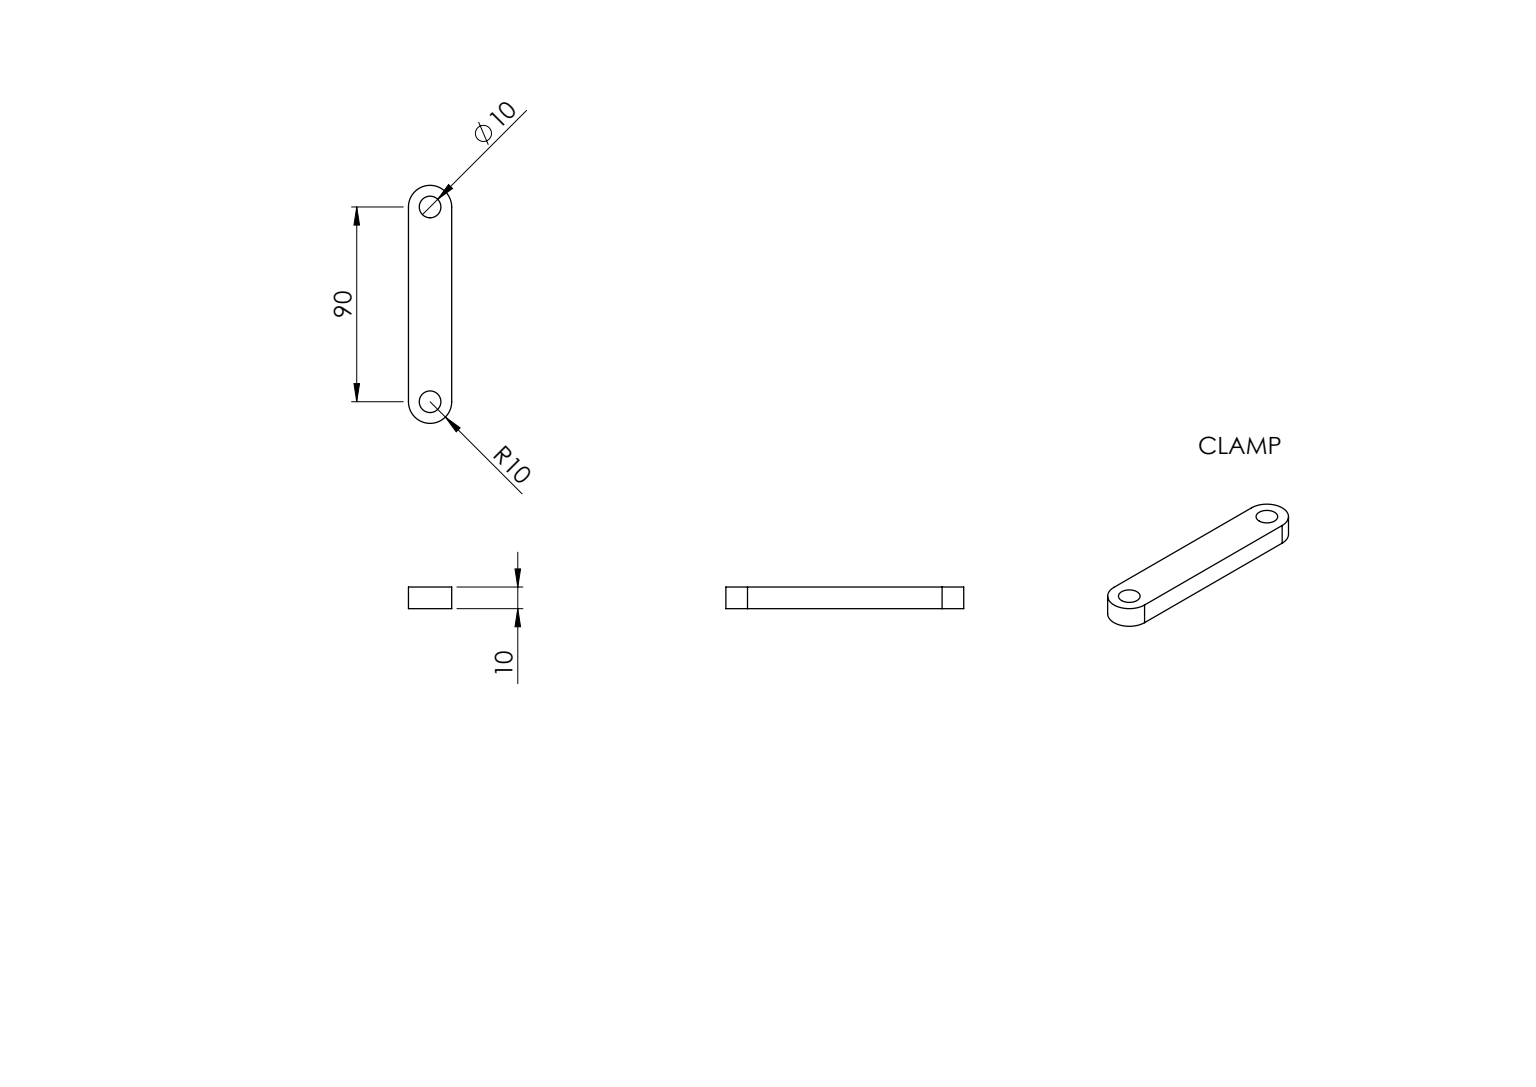
ISO-10303-21;
HEADER;
FILE_DESCRIPTION (('STEP AP214'),
    '1' );
FILE_NAME ('clamp.step',
    '2026-10-27T14:18:53',
    ( '' ),
    ( '' ),
    'SwSTEP 2.0',
    'SolidWorks 2026',
    '' );
FILE_SCHEMA (( 'AUTOMOTIVE_DESIGN' ));
ENDSEC;

DATA;
#13=EDGE_LOOP ( 'NONE', ( #5766, #2705, #5746, #232 ) ) ;
#85=ORIENTED_EDGE ( 'NONE', *, *, #3683, .T. ) ;
#87=DIRECTION ( 'NONE',  ( -0.000000000000000000, -1.000000000000000000, -0.000000000000000000 ) ) ;
#88=CIRCLE ( 'NONE', #5797, 5.000000000000004441 ) ;
#89=CARTESIAN_POINT ( 'NONE',  ( -55.00000000000001421, 40.00000000000000000, -45.00000000000000000 ) ) ;
#105=VERTEX_POINT ( 'NONE', #4634 ) ;
#111=VERTEX_POINT ( 'NONE', #3686 ) ;
#120=FACE_BOUND ( 'NONE', #3180, .T. ) ;
#147=CLOSED_SHELL ( 'NONE', ( #248, #2661, #5068, #1341, #3720, #5571, #3327, #1429, #4479, #1422, #4024 ) ) ;
#150=DIRECTION ( 'NONE',  ( 0.000000000000000000, 1.000000000000000000, 0.000000000000000000 ) ) ;
#188=STYLED_ITEM('',(#6006),#2182);
#203=EDGE_CURVE ( 'NONE', #1147, #2495, #5910, .T. ) ;
#217=ORIENTED_EDGE ( 'NONE', *, *, #5542, .F. ) ;
#232=ORIENTED_EDGE ( 'NONE', *, *, #1791, .F. ) ;
#234=DIRECTION ( 'NONE',  ( 0.000000000000000000, 1.000000000000000000, 0.000000000000000000 ) ) ;
#248=ADVANCED_FACE ( 'NONE', ( #4015 ), #1620, .F. ) ;
#256=APPLICATION_CONTEXT ( 'automotive_design' ) ;
#258=ORIENTED_EDGE ( 'NONE', *, *, #3702, .T. ) ;
#270=DIRECTION ( 'NONE',  ( -0.000000000000000000, -1.000000000000000000, -0.000000000000000000 ) ) ;
#325=CARTESIAN_POINT ( 'NONE',  ( -45.00000000000001421, 30.00000000000000355, -50.00000000000000000 ) ) ;
#340=LINE ( 'NONE', #5874, #5255 ) ;
#355=CARTESIAN_POINT ( 'NONE',  ( -45.00000000000001421, 40.00000000000000000, 50.00000000000000000 ) ) ;
#361=AXIS2_PLACEMENT_3D ( 'NONE', #2845, #4273, #538 ) ;
#367=EDGE_CURVE ( 'NONE', #1773, #5556, #4512, .T. ) ;
#377=VERTEX_POINT ( 'NONE', #441 ) ;
#417=VECTOR ( 'NONE', #1999, 1000.000000000000000 ) ;
#441=CARTESIAN_POINT ( 'NONE',  ( -45.00000000000001421, 40.00000000000000000, 50.00000000000000000 ) ) ;
#531=EDGE_CURVE ( 'NONE', #1773, #105, #641, .T. ) ;
#538=DIRECTION ( 'NONE',  ( 0.000000000000000000, 0.000000000000000000, -1.000000000000000000 ) ) ;
#569=ORIENTED_EDGE ( 'NONE', *, *, #1573, .F. ) ;
#596=PRODUCT_CONTEXT ( 'NONE', #256, 'mechanical' ) ;
#608=( NAMED_UNIT ( * ) PLANE_ANGLE_UNIT ( ) SI_UNIT ( $, .RADIAN. ) );
#625=DIRECTION ( 'NONE',  ( -0.000000000000000000, -1.000000000000000000, -0.000000000000000000 ) ) ;
#641=LINE ( 'NONE', #2484, #4530 ) ;
#649=DIRECTION ( 'NONE',  ( 0.000000000000000000, 0.000000000000000000, 1.000000000000000000 ) ) ;
#657=DIRECTION ( 'NONE',  ( 0.000000000000000000, 0.000000000000000000, 1.000000000000000000 ) ) ;
#667=DIRECTION ( 'NONE',  ( 1.000000000000000000, 0.000000000000000000, 0.000000000000000000 ) ) ;
#716=CARTESIAN_POINT ( 'NONE',  ( -45.00000000000001421, 40.00000000000000000, -55.00000000000000000 ) ) ;
#719=EDGE_CURVE ( 'NONE', #4755, #3109, #5913, .T. ) ;
#720=CARTESIAN_POINT ( 'NONE',  ( -45.00000000000001421, 40.00000000000000000, -45.00000000000000000 ) ) ;
#739=ORIENTED_EDGE ( 'NONE', *, *, #1238, .F. ) ;
#747=PLANE ( 'NONE',  #3499 ) ;
#791=PRODUCT_DEFINITION ( 'UNKNOWN', '', #4303, #1117 ) ;
#796=EDGE_LOOP ( 'NONE', ( #4911, #5822 ) ) ;
#813=CARTESIAN_POINT ( 'NONE',  ( -35.00000000000000711, 30.00000000000000355, 45.00000000000000000 ) ) ;
#840=DIRECTION ( 'NONE',  ( 0.000000000000000000, 1.000000000000000000, 0.000000000000000000 ) ) ;
#842=DIRECTION ( 'NONE',  ( 0.000000000000000000, 0.000000000000000000, -1.000000000000000000 ) ) ;
#858=CARTESIAN_POINT ( 'NONE',  ( -45.00000000000001421, 40.00000000000000000, 45.00000000000000000 ) ) ;
#869=FACE_OUTER_BOUND ( 'NONE', #5036, .T. ) ;
#908=DIRECTION ( 'NONE',  ( 0.000000000000000000, 0.000000000000000000, 1.000000000000000000 ) ) ;
#939=VERTEX_POINT ( 'NONE', #5636 ) ;
#955=ORIENTED_EDGE ( 'NONE', *, *, #1985, .T. ) ;
#956=MECHANICAL_DESIGN_GEOMETRIC_PRESENTATION_REPRESENTATION('',(#188),#1645);
#995=FACE_OUTER_BOUND ( 'NONE', #13, .T. ) ;
#996=DIRECTION ( 'NONE',  ( 0.000000000000000000, 0.000000000000000000, 1.000000000000000000 ) ) ;
#1011=ORIENTED_EDGE ( 'NONE', *, *, #1756, .T. ) ;
#1018=EDGE_LOOP ( 'NONE', ( #5388, #1028, #3124, #4232 ) ) ;
#1028=ORIENTED_EDGE ( 'NONE', *, *, #5949, .F. ) ;
#1048=ORIENTED_EDGE ( 'NONE', *, *, #3427, .F. ) ;
#1057=AXIS2_PLACEMENT_3D ( 'NONE', #1923, #4598, #1476 ) ;
#1101=FACE_OUTER_BOUND ( 'NONE', #4420, .T. ) ;
#1113=SHAPE_REPRESENTATION ( 'clamp', ( #5080 ), #4776 ) ;
#1116=UNCERTAINTY_MEASURE_WITH_UNIT (LENGTH_MEASURE( 1.000000000000000082E-05 ), #1219, 'distance_accuracy_value', 'NONE');
#1117=PRODUCT_DEFINITION_CONTEXT ( 'detailed design', #5329, 'design' ) ;
#1120=EDGE_CURVE ( 'NONE', #3568, #3307, #2068, .T. ) ;
#1134=LINE ( 'NONE', #2938, #3781 ) ;
#1147=VERTEX_POINT ( 'NONE', #4828 ) ;
#1159=AXIS2_PLACEMENT_3D ( 'NONE', #3827, #1520, #5224 ) ;
#1190=( NAMED_UNIT ( * ) SI_UNIT ( $, .STERADIAN. ) SOLID_ANGLE_UNIT ( ) );
#1193=DIRECTION ( 'NONE',  ( -1.000000000000000000, 0.000000000000000000, 0.000000000000000000 ) ) ;
#1215=CARTESIAN_POINT ( 'NONE',  ( -55.00000000000001421, 30.00000000000000355, -45.00000000000000000 ) ) ;
#1219=( LENGTH_UNIT ( ) NAMED_UNIT ( * ) SI_UNIT ( .MILLI., .METRE. ) );
#1222=CARTESIAN_POINT ( 'NONE',  ( -35.00000000000000711, 40.00000000000000000, 45.00000000000000000 ) ) ;
#1230=CARTESIAN_POINT ( 'NONE',  ( -45.00000000000001421, 30.00000000000000355, -45.00000000000000000 ) ) ;
#1238=EDGE_CURVE ( 'NONE', #3109, #3549, #5477, .T. ) ;
#1257=ORIENTED_EDGE ( 'NONE', *, *, #1573, .T. ) ;
#1273=VECTOR ( 'NONE', #2528, 1000.000000000000000 ) ;
#1276=FILL_AREA_STYLE ('',( #3580 ) ) ;
#1287=EDGE_CURVE ( 'NONE', #2495, #4600, #3639, .T. ) ;
#1298=DIRECTION ( 'NONE',  ( -0.000000000000000000, -1.000000000000000000, -0.000000000000000000 ) ) ;
#1301=CARTESIAN_POINT ( 'NONE',  ( -45.00000000000001421, 40.00000000000000000, 45.00000000000000000 ) ) ;
#1341=ADVANCED_FACE ( 'NONE', ( #2873, #5209, #120 ), #1898, .T. ) ;
#1349=DIRECTION ( 'NONE',  ( 0.000000000000000000, 1.000000000000000000, 0.000000000000000000 ) ) ;
#1358=ORIENTED_EDGE ( 'NONE', *, *, #203, .T. ) ;
#1362=DIRECTION ( 'NONE',  ( -0.000000000000000000, -0.000000000000000000, 1.000000000000000000 ) ) ;
#1368=AXIS2_PLACEMENT_3D ( 'NONE', #858, #3655, #4231 ) ;
#1380=VECTOR ( 'NONE', #2853, 1000.000000000000000 ) ;
#1418=CIRCLE ( 'NONE', #2117, 10.00000000000000178 ) ;
#1422=ADVANCED_FACE ( 'NONE', ( #995 ), #3810, .F. ) ;
#1425=CARTESIAN_POINT ( 'NONE',  ( -45.00000000000001421, 40.00000000000000000, -45.00000000000000000 ) ) ;
#1429=ADVANCED_FACE ( 'NONE', ( #2386 ), #1532, .T. ) ;
#1476=DIRECTION ( 'NONE',  ( 0.000000000000000000, 0.000000000000000000, -1.000000000000000000 ) ) ;
#1493=ORIENTED_EDGE ( 'NONE', *, *, #1238, .T. ) ;
#1495=AXIS2_PLACEMENT_3D ( 'NONE', #1301, #2761, #908 ) ;
#1520=DIRECTION ( 'NONE',  ( 0.000000000000000000, 1.000000000000000000, 0.000000000000000000 ) ) ;
#1532=CYLINDRICAL_SURFACE ( 'NONE', #5018, 10.00000000000000178 ) ;
#1559=CIRCLE ( 'NONE', #5347, 10.00000000000000178 ) ;
#1573=EDGE_CURVE ( 'NONE', #939, #3970, #2780, .T. ) ;
#1607=UNCERTAINTY_MEASURE_WITH_UNIT (LENGTH_MEASURE( 1.000000000000000082E-05 ), #5602, 'distance_accuracy_value', 'NONE');
#1609=ORIENTED_EDGE ( 'NONE', *, *, #4675, .T. ) ;
#1620=CYLINDRICAL_SURFACE ( 'NONE', #5826, 5.000000000000004441 ) ;
#1633=DIRECTION ( 'NONE',  ( 0.000000000000000000, 0.000000000000000000, 1.000000000000000000 ) ) ;
#1638=DIRECTION ( 'NONE',  ( 0.000000000000000000, 0.000000000000000000, 1.000000000000000000 ) ) ;
#1640=AXIS2_PLACEMENT_3D ( 'NONE', #1230, #1744, #3085 ) ;
#1645=( GEOMETRIC_REPRESENTATION_CONTEXT ( 3 ) GLOBAL_UNCERTAINTY_ASSIGNED_CONTEXT ( ( #1116 ) ) GLOBAL_UNIT_ASSIGNED_CONTEXT ( ( #1219, #1735, #1190 ) ) REPRESENTATION_CONTEXT ( 'NONE', 'WORKASPACE' ) );
#1657=AXIS2_PLACEMENT_3D ( 'NONE', #3859, #1193, #2931 ) ;
#1658=EDGE_LOOP ( 'NONE', ( #1048, #3597, #2673, #5918 ) ) ;
#1659=EDGE_CURVE ( 'NONE', #111, #377, #88, .T. ) ;
#1663=DIRECTION ( 'NONE',  ( 0.000000000000000000, 0.000000000000000000, 1.000000000000000000 ) ) ;
#1683=ORIENTED_EDGE ( 'NONE', *, *, #3427, .T. ) ;
#1691=CARTESIAN_POINT ( 'NONE',  ( -35.00000000000000711, 40.00000000000000000, -45.00000000000000000 ) ) ;
#1694=DIRECTION ( 'NONE',  ( -0.000000000000000000, -1.000000000000000000, -0.000000000000000000 ) ) ;
#1723=EDGE_CURVE ( 'NONE', #3307, #3568, #2735, .T. ) ;
#1735=( NAMED_UNIT ( * ) PLANE_ANGLE_UNIT ( ) SI_UNIT ( $, .RADIAN. ) );
#1744=DIRECTION ( 'NONE',  ( 0.000000000000000000, 1.000000000000000000, 0.000000000000000000 ) ) ;
#1748=CYLINDRICAL_SURFACE ( 'NONE', #3511, 10.00000000000000178 ) ;
#1756=EDGE_CURVE ( 'NONE', #5556, #4755, #1418, .T. ) ;
#1773=VERTEX_POINT ( 'NONE', #1691 ) ;
#1786=ORIENTED_EDGE ( 'NONE', *, *, #203, .F. ) ;
#1791=EDGE_CURVE ( 'NONE', #3262, #2126, #4120, .T. ) ;
#1811=EDGE_LOOP ( 'NONE', ( #569, #4895 ) ) ;
#1853=DIRECTION ( 'NONE',  ( 0.000000000000000000, 0.000000000000000000, 1.000000000000000000 ) ) ;
#1898=PLANE ( 'NONE',  #5578 ) ;
#1915=CARTESIAN_POINT ( 'NONE',  ( -55.00000000000001421, 40.00000000000000000, 45.00000000000000000 ) ) ;
#1921=DIRECTION ( 'NONE',  ( 0.000000000000000000, 0.000000000000000000, -1.000000000000000000 ) ) ;
#1923=CARTESIAN_POINT ( 'NONE',  ( -45.00000000000001421, 40.00000000000000000, -45.00000000000000000 ) ) ;
#1927=PRODUCT ( 'clamp', 'clamp', '', ( #596 ) ) ;
#1929=( NAMED_UNIT ( * ) SI_UNIT ( $, .STERADIAN. ) SOLID_ANGLE_UNIT ( ) );
#1985=EDGE_CURVE ( 'NONE', #4600, #2954, #2800, .T. ) ;
#1999=DIRECTION ( 'NONE',  ( -0.000000000000000000, -1.000000000000000000, -0.000000000000000000 ) ) ;
#2008=PLANE ( 'NONE',  #1657 ) ;
#2011=EDGE_LOOP ( 'NONE', ( #5869, #5688, #1358, #5895 ) ) ;
#2014=FACE_BOUND ( 'NONE', #796, .T. ) ;
#2033=ORIENTED_EDGE ( 'NONE', *, *, #4675, .F. ) ;
#2054=( GEOMETRIC_REPRESENTATION_CONTEXT ( 3 ) GLOBAL_UNCERTAINTY_ASSIGNED_CONTEXT ( ( #1607 ) ) GLOBAL_UNIT_ASSIGNED_CONTEXT ( ( #5602, #608, #1929 ) ) REPRESENTATION_CONTEXT ( 'NONE', 'WORKASPACE' ) );
#2055=CARTESIAN_POINT ( 'NONE',  ( -55.00000000000001421, 30.00000000000000355, 45.00000000000000000 ) ) ;
#2068=CIRCLE ( 'NONE', #2945, 5.000000000000004441 ) ;
#2082=FACE_BOUND ( 'NONE', #2783, .T. ) ;
#2085=DIRECTION ( 'NONE',  ( 0.000000000000000000, 1.000000000000000000, 0.000000000000000000 ) ) ;
#2117=AXIS2_PLACEMENT_3D ( 'NONE', #3634, #840, #2175 ) ;
#2126=VERTEX_POINT ( 'NONE', #325 ) ;
#2139=VECTOR ( 'NONE', #3110, 1000.000000000000000 ) ;
#2143=CARTESIAN_POINT ( 'NONE',  ( -55.00000000000001421, 40.00000000000000000, -45.00000000000000000 ) ) ;
#2154=COLOUR_RGB ( '',0.8941176470588234615, 0.8941176470588234615, 0.8941176470588234615 ) ;
#2175=DIRECTION ( 'NONE',  ( 0.000000000000000000, 0.000000000000000000, 1.000000000000000000 ) ) ;
#2182=MANIFOLD_SOLID_BREP ( 'Boss-Extrude1', #147 ) ;
#2185=( NAMED_UNIT ( * ) PLANE_ANGLE_UNIT ( ) SI_UNIT ( $, .RADIAN. ) );
#2221=LINE ( 'NONE', #355, #2139 ) ;
#2229=DIRECTION ( 'NONE',  ( 0.000000000000000000, 0.000000000000000000, 1.000000000000000000 ) ) ;
#2342=MECHANICAL_DESIGN_GEOMETRIC_PRESENTATION_REPRESENTATION('',(#5551),#2054);
#2386=FACE_OUTER_BOUND ( 'NONE', #5197, .T. ) ;
#2437=AXIS2_PLACEMENT_3D ( 'NONE', #5011, #5511, #2718 ) ;
#2452=EDGE_LOOP ( 'NONE', ( #5202, #4313, #1786, #5741, #3673 ) ) ;
#2468=LINE ( 'NONE', #3416, #4285 ) ;
#2484=CARTESIAN_POINT ( 'NONE',  ( -35.00000000000000711, 40.00000000000000000, -45.00000000000000000 ) ) ;
#2494=FACE_OUTER_BOUND ( 'NONE', #2011, .T. ) ;
#2495=VERTEX_POINT ( 'NONE', #1215 ) ;
#2528=DIRECTION ( 'NONE',  ( 0.000000000000000000, 0.000000000000000000, -1.000000000000000000 ) ) ;
#2538=DIRECTION ( 'NONE',  ( 0.000000000000000000, 0.000000000000000000, -1.000000000000000000 ) ) ;
#2613=CARTESIAN_POINT ( 'NONE',  ( -45.00000000000001421, 40.00000000000000000, 45.00000000000000000 ) ) ;
#2641=AXIS2_PLACEMENT_3D ( 'NONE', #4733, #5664, #5632 ) ;
#2661=ADVANCED_FACE ( 'NONE', ( #5210 ), #2904, .F. ) ;
#2673=ORIENTED_EDGE ( 'NONE', *, *, #5542, .T. ) ;
#2696=DIRECTION ( 'NONE',  ( -0.000000000000000000, -0.000000000000000000, 1.000000000000000000 ) ) ;
#2705=ORIENTED_EDGE ( 'NONE', *, *, #2725, .T. ) ;
#2718=DIRECTION ( 'NONE',  ( 0.000000000000000000, 0.000000000000000000, 1.000000000000000000 ) ) ;
#2725=EDGE_CURVE ( 'NONE', #3970, #939, #4851, .T. ) ;
#2735=CIRCLE ( 'NONE', #2437, 5.000000000000004441 ) ;
#2761=DIRECTION ( 'NONE',  ( 0.000000000000000000, 1.000000000000000000, 0.000000000000000000 ) ) ;
#2780=CIRCLE ( 'NONE', #3556, 5.000000000000004441 ) ;
#2783=EDGE_LOOP ( 'NONE', ( #1609, #3056 ) ) ;
#2791=EDGE_CURVE ( 'NONE', #4755, #2495, #4562, .T. ) ;
#2800=CIRCLE ( 'NONE', #5416, 10.00000000000000178 ) ;
#2845=CARTESIAN_POINT ( 'NONE',  ( -45.00000000000001421, 40.00000000000000000, -45.00000000000000000 ) ) ;
#2853=DIRECTION ( 'NONE',  ( -0.000000000000000000, -1.000000000000000000, -0.000000000000000000 ) ) ;
#2873=FACE_BOUND ( 'NONE', #1811, .T. ) ;
#2896=CARTESIAN_POINT ( 'NONE',  ( -45.00000000000001421, 40.00000000000000000, -45.00000000000000000 ) ) ;
#2904=CYLINDRICAL_SURFACE ( 'NONE', #1057, 5.000000000000004441 ) ;
#2910=PRESENTATION_STYLE_ASSIGNMENT (( #4767 ) ) ;
#2931=DIRECTION ( 'NONE',  ( 0.000000000000000000, 0.000000000000000000, 1.000000000000000000 ) ) ;
#2938=CARTESIAN_POINT ( 'NONE',  ( -35.00000000000000711, 40.00000000000000000, 45.00000000000000000 ) ) ;
#2945=AXIS2_PLACEMENT_3D ( 'NONE', #4949, #3938, #1638 ) ;
#2954=VERTEX_POINT ( 'NONE', #813 ) ;
#2955=ORIENTED_EDGE ( 'NONE', *, *, #531, .F. ) ;
#2994=VECTOR ( 'NONE', #1362, 1000.000000000000000 ) ;
#2995=CARTESIAN_POINT ( 'NONE',  ( -45.00000000000001421, 30.00000000000000355, -45.00000000000000000 ) ) ;
#3006=VECTOR ( 'NONE', #3197, 1000.000000000000000 ) ;
#3021=CARTESIAN_POINT ( 'NONE',  ( -45.00000000000001421, 30.00000000000000355, -39.99999999999999289 ) ) ;
#3022=CARTESIAN_POINT ( 'NONE',  ( -45.00000000000001421, 40.00000000000000000, 45.00000000000000000 ) ) ;
#3056=ORIENTED_EDGE ( 'NONE', *, *, #1791, .T. ) ;
#3068=CARTESIAN_POINT ( 'NONE',  ( -45.00000000000001421, 40.00000000000000000, -39.99999999999999289 ) ) ;
#3075=ORIENTED_EDGE ( 'NONE', *, *, #1659, .T. ) ;
#3085=DIRECTION ( 'NONE',  ( 0.000000000000000000, 0.000000000000000000, 1.000000000000000000 ) ) ;
#3109=VERTEX_POINT ( 'NONE', #1915 ) ;
#3110=DIRECTION ( 'NONE',  ( -0.000000000000000000, -1.000000000000000000, -0.000000000000000000 ) ) ;
#3124=ORIENTED_EDGE ( 'NONE', *, *, #719, .F. ) ;
#3126=AXIS2_PLACEMENT_3D ( 'NONE', #3022, #4880, #3508 ) ;
#3135=SURFACE_STYLE_FILL_AREA ( #1276 ) ;
#3180=EDGE_LOOP ( 'NONE', ( #4513, #3847 ) ) ;
#3195=( NAMED_UNIT ( * ) SI_UNIT ( $, .STERADIAN. ) SOLID_ANGLE_UNIT ( ) );
#3197=DIRECTION ( 'NONE',  ( -0.000000000000000000, -1.000000000000000000, -0.000000000000000000 ) ) ;
#3215=CARTESIAN_POINT ( 'NONE',  ( -45.00000000000001421, 40.00000000000000000, 45.00000000000000000 ) ) ;
#3257=CARTESIAN_POINT ( 'NONE',  ( -55.00000000000001421, 40.00000000000000000, 45.00000000000000000 ) ) ;
#3262=VERTEX_POINT ( 'NONE', #3021 ) ;
#3303=DIRECTION ( 'NONE',  ( 0.000000000000000000, 1.000000000000000000, 0.000000000000000000 ) ) ;
#3307=VERTEX_POINT ( 'NONE', #5361 ) ;
#3327=ADVANCED_FACE ( 'NONE', ( #1101 ), #2008, .F. ) ;
#3362=CARTESIAN_POINT ( 'NONE',  ( -45.00000000000001421, 40.00000000000000000, -45.00000000000000000 ) ) ;
#3416=CARTESIAN_POINT ( 'NONE',  ( -45.00000000000001421, 40.00000000000000000, -50.00000000000000000 ) ) ;
#3427=EDGE_CURVE ( 'NONE', #377, #3307, #2221, .T. ) ;
#3499=AXIS2_PLACEMENT_3D ( 'NONE', #4308, #150, #3838 ) ;
#3504=AXIS2_PLACEMENT_3D ( 'NONE', #2896, #4786, #4816 ) ;
#3508=DIRECTION ( 'NONE',  ( 0.000000000000000000, 0.000000000000000000, -1.000000000000000000 ) ) ;
#3511=AXIS2_PLACEMENT_3D ( 'NONE', #4430, #270, #842 ) ;
#3516=CARTESIAN_POINT ( 'NONE',  ( -35.00000000000000711, 40.00000000000000000, 45.00000000000000000 ) ) ;
#3527=CARTESIAN_POINT ( 'NONE',  ( 0.000000000000000000, 0.000000000000000000, 0.000000000000000000 ) ) ;
#3549=VERTEX_POINT ( 'NONE', #1222 ) ;
#3556=AXIS2_PLACEMENT_3D ( 'NONE', #720, #5811, #657 ) ;
#3565=CARTESIAN_POINT ( 'NONE',  ( -45.00000000000001421, 40.00000000000000000, -39.99999999999999289 ) ) ;
#3568=VERTEX_POINT ( 'NONE', #4608 ) ;
#3580=FILL_AREA_STYLE_COLOUR ( '', #2154 ) ;
#3597=ORIENTED_EDGE ( 'NONE', *, *, #4048, .T. ) ;
#3599=VECTOR ( 'NONE', #625, 1000.000000000000000 ) ;
#3634=CARTESIAN_POINT ( 'NONE',  ( -45.00000000000001421, 40.00000000000000000, -45.00000000000000000 ) ) ;
#3639=LINE ( 'NONE', #4057, #5461 ) ;
#3655=DIRECTION ( 'NONE',  ( 0.000000000000000000, 1.000000000000000000, 0.000000000000000000 ) ) ;
#3673=ORIENTED_EDGE ( 'NONE', *, *, #3755, .F. ) ;
#3683=EDGE_CURVE ( 'NONE', #3549, #1773, #1134, .T. ) ;
#3686=CARTESIAN_POINT ( 'NONE',  ( -45.00000000000001421, 40.00000000000000000, 39.99999999999999289 ) ) ;
#3702=EDGE_CURVE ( 'NONE', #105, #1147, #1559, .T. ) ;
#3720=ADVANCED_FACE ( 'NONE', ( #4917, #2082, #2014 ), #747, .F. ) ;
#3755=EDGE_CURVE ( 'NONE', #2954, #105, #5711, .T. ) ;
#3778=PLANE ( 'NONE',  #2641 ) ;
#3781=VECTOR ( 'NONE', #2538, 1000.000000000000000 ) ;
#3789=ORIENTED_EDGE ( 'NONE', *, *, #3683, .F. ) ;
#3803=ORIENTED_EDGE ( 'NONE', *, *, #4249, .T. ) ;
#3807=LINE ( 'NONE', #716, #3599 ) ;
#3810=CYLINDRICAL_SURFACE ( 'NONE', #361, 5.000000000000004441 ) ;
#3814=ORIENTED_EDGE ( 'NONE', *, *, #5105, .F. ) ;
#3826=EDGE_CURVE ( 'NONE', #939, #2126, #2468, .T. ) ;
#3827=CARTESIAN_POINT ( 'NONE',  ( -45.00000000000001421, 30.00000000000000355, -45.00000000000000000 ) ) ;
#3838=DIRECTION ( 'NONE',  ( 0.000000000000000000, -0.000000000000000000, 1.000000000000000000 ) ) ;
#3847=ORIENTED_EDGE ( 'NONE', *, *, #4048, .F. ) ;
#3859=CARTESIAN_POINT ( 'NONE',  ( -35.00000000000000711, 40.00000000000000000, 45.00000000000000000 ) ) ;
#3938=DIRECTION ( 'NONE',  ( 0.000000000000000000, 1.000000000000000000, 0.000000000000000000 ) ) ;
#3954=FACE_OUTER_BOUND ( 'NONE', #1658, .T. ) ;
#3970=VERTEX_POINT ( 'NONE', #3565 ) ;
#4015=FACE_OUTER_BOUND ( 'NONE', #4948, .T. ) ;
#4024=ADVANCED_FACE ( 'NONE', ( #3954 ), #5807, .F. ) ;
#4028=CARTESIAN_POINT ( 'NONE',  ( -45.00000000000001421, 40.00000000000000000, -55.00000000000000000 ) ) ;
#4048=EDGE_CURVE ( 'NONE', #377, #111, #5733, .T. ) ;
#4057=CARTESIAN_POINT ( 'NONE',  ( -55.00000000000001421, 30.00000000000000355, 45.00000000000000000 ) ) ;
#4120=CIRCLE ( 'NONE', #1640, 5.000000000000004441 ) ;
#4219=DIRECTION ( 'NONE',  ( 0.000000000000000000, 1.000000000000000000, 0.000000000000000000 ) ) ;
#4222=PRODUCT_DEFINITION_SHAPE ( 'NONE', 'NONE',  #791 ) ;
#4223=ORIENTED_EDGE ( 'NONE', *, *, #367, .F. ) ;
#4231=DIRECTION ( 'NONE',  ( 0.000000000000000000, 0.000000000000000000, 1.000000000000000000 ) ) ;
#4232=ORIENTED_EDGE ( 'NONE', *, *, #2791, .T. ) ;
#4249=EDGE_CURVE ( 'NONE', #3970, #3262, #4900, .T. ) ;
#4263=ORIENTED_EDGE ( 'NONE', *, *, #5574, .T. ) ;
#4273=DIRECTION ( 'NONE',  ( -0.000000000000000000, -1.000000000000000000, -0.000000000000000000 ) ) ;
#4285=VECTOR ( 'NONE', #4332, 1000.000000000000000 ) ;
#4288=LINE ( 'NONE', #4739, #1380 ) ;
#4302=CARTESIAN_POINT ( 'NONE',  ( -35.00000000000000711, 30.00000000000000355, 45.00000000000000000 ) ) ;
#4303=PRODUCT_DEFINITION_FORMATION_WITH_SPECIFIED_SOURCE ( 'ANY', '', #1927, .NOT_KNOWN. ) ;
#4306=SHAPE_DEFINITION_REPRESENTATION ( #4222, #1113 ) ;
#4308=CARTESIAN_POINT ( 'NONE',  ( -45.00000000000001421, 30.00000000000000355, 45.00000000000000000 ) ) ;
#4313=ORIENTED_EDGE ( 'NONE', *, *, #1287, .F. ) ;
#4330=ORIENTED_EDGE ( 'NONE', *, *, #5574, .F. ) ;
#4332=DIRECTION ( 'NONE',  ( -0.000000000000000000, -1.000000000000000000, -0.000000000000000000 ) ) ;
#4376=CIRCLE ( 'NONE', #4875, 5.000000000000004441 ) ;
#4420=EDGE_LOOP ( 'NONE', ( #5901, #2955, #3789, #4263 ) ) ;
#4430=CARTESIAN_POINT ( 'NONE',  ( -45.00000000000001421, 40.00000000000000000, 45.00000000000000000 ) ) ;
#4478=DIRECTION ( 'NONE',  ( 0.000000000000000000, 0.000000000000000000, -1.000000000000000000 ) ) ;
#4479=ADVANCED_FACE ( 'NONE', ( #5553 ), #3778, .F. ) ;
#4489=VECTOR ( 'NONE', #1694, 1000.000000000000000 ) ;
#4512=CIRCLE ( 'NONE', #5490, 10.00000000000000178 ) ;
#4513=ORIENTED_EDGE ( 'NONE', *, *, #1659, .F. ) ;
#4530=VECTOR ( 'NONE', #5195, 1000.000000000000000 ) ;
#4562=LINE ( 'NONE', #89, #3006 ) ;
#4596=( LENGTH_UNIT ( ) NAMED_UNIT ( * ) SI_UNIT ( .MILLI., .METRE. ) );
#4598=DIRECTION ( 'NONE',  ( -0.000000000000000000, -1.000000000000000000, -0.000000000000000000 ) ) ;
#4600=VERTEX_POINT ( 'NONE', #2055 ) ;
#4603=DIRECTION ( 'NONE',  ( 0.000000000000000000, 1.000000000000000000, 0.000000000000000000 ) ) ;
#4608=CARTESIAN_POINT ( 'NONE',  ( -45.00000000000001421, 30.00000000000000355, 39.99999999999999289 ) ) ;
#4634=CARTESIAN_POINT ( 'NONE',  ( -35.00000000000000711, 30.00000000000000355, -45.00000000000000000 ) ) ;
#4675=EDGE_CURVE ( 'NONE', #2126, #3262, #4376, .T. ) ;
#4733=CARTESIAN_POINT ( 'NONE',  ( -55.00000000000001421, 40.00000000000000000, 45.00000000000000000 ) ) ;
#4739=CARTESIAN_POINT ( 'NONE',  ( -55.00000000000001421, 40.00000000000000000, 45.00000000000000000 ) ) ;
#4755=VERTEX_POINT ( 'NONE', #2143 ) ;
#4757=CARTESIAN_POINT ( 'NONE',  ( -45.00000000000001421, 40.00000000000000000, 45.00000000000000000 ) ) ;
#4767=SURFACE_STYLE_USAGE ( .BOTH. , #4993 ) ;
#4776=( GEOMETRIC_REPRESENTATION_CONTEXT ( 3 ) GLOBAL_UNCERTAINTY_ASSIGNED_CONTEXT ( ( #5670 ) ) GLOBAL_UNIT_ASSIGNED_CONTEXT ( ( #4596, #2185, #3195 ) ) REPRESENTATION_CONTEXT ( 'NONE', 'WORKASPACE' ) );
#4786=DIRECTION ( 'NONE',  ( -0.000000000000000000, -1.000000000000000000, -0.000000000000000000 ) ) ;
#4816=DIRECTION ( 'NONE',  ( 0.000000000000000000, 0.000000000000000000, -1.000000000000000000 ) ) ;
#4828=CARTESIAN_POINT ( 'NONE',  ( -45.00000000000001421, 30.00000000000000355, -55.00000000000000000 ) ) ;
#4831=DIRECTION ( 'NONE',  ( 0.000000000000000000, 0.000000000000000000, 1.000000000000000000 ) ) ;
#4850=DIRECTION ( 'NONE',  ( 0.000000000000000000, 1.000000000000000000, 0.000000000000000000 ) ) ;
#4851=CIRCLE ( 'NONE', #5813, 5.000000000000004441 ) ;
#4875=AXIS2_PLACEMENT_3D ( 'NONE', #5243, #2085, #1633 ) ;
#4880=DIRECTION ( 'NONE',  ( -0.000000000000000000, -1.000000000000000000, -0.000000000000000000 ) ) ;
#4895=ORIENTED_EDGE ( 'NONE', *, *, #2725, .F. ) ;
#4900=LINE ( 'NONE', #3068, #417 ) ;
#4911=ORIENTED_EDGE ( 'NONE', *, *, #1120, .T. ) ;
#4917=FACE_OUTER_BOUND ( 'NONE', #2452, .T. ) ;
#4932=ORIENTED_EDGE ( 'NONE', *, *, #719, .T. ) ;
#4948=EDGE_LOOP ( 'NONE', ( #3075, #1683, #5771, #217 ) ) ;
#4949=CARTESIAN_POINT ( 'NONE',  ( -45.00000000000001421, 30.00000000000000355, 45.00000000000000000 ) ) ;
#4993=SURFACE_SIDE_STYLE ('',( #3135 ) ) ;
#5011=CARTESIAN_POINT ( 'NONE',  ( -45.00000000000001421, 30.00000000000000355, 45.00000000000000000 ) ) ;
#5018=AXIS2_PLACEMENT_3D ( 'NONE', #3362, #87, #1921 ) ;
#5036=EDGE_LOOP ( 'NONE', ( #955, #4330, #739, #5709 ) ) ;
#5068=ADVANCED_FACE ( 'NONE', ( #2494 ), #5713, .T. ) ;
#5080=AXIS2_PLACEMENT_3D ( 'NONE', #3527, #4831, #667 ) ;
#5105=EDGE_CURVE ( 'NONE', #5556, #1147, #3807, .T. ) ;
#5135=ORIENTED_EDGE ( 'NONE', *, *, #3826, .F. ) ;
#5174=ORIENTED_EDGE ( 'NONE', *, *, #367, .T. ) ;
#5195=DIRECTION ( 'NONE',  ( -0.000000000000000000, -1.000000000000000000, -0.000000000000000000 ) ) ;
#5197=EDGE_LOOP ( 'NONE', ( #3814, #4223, #5275, #258 ) ) ;
#5202=ORIENTED_EDGE ( 'NONE', *, *, #1985, .F. ) ;
#5209=FACE_OUTER_BOUND ( 'NONE', #5373, .T. ) ;
#5210=FACE_OUTER_BOUND ( 'NONE', #5925, .T. ) ;
#5224=DIRECTION ( 'NONE',  ( 0.000000000000000000, 0.000000000000000000, 1.000000000000000000 ) ) ;
#5243=CARTESIAN_POINT ( 'NONE',  ( -45.00000000000001421, 30.00000000000000355, -45.00000000000000000 ) ) ;
#5255=VECTOR ( 'NONE', #1298, 1000.000000000000000 ) ;
#5275=ORIENTED_EDGE ( 'NONE', *, *, #531, .T. ) ;
#5329=APPLICATION_CONTEXT ( 'automotive_design' ) ;
#5347=AXIS2_PLACEMENT_3D ( 'NONE', #2995, #4850, #1663 ) ;
#5361=CARTESIAN_POINT ( 'NONE',  ( -45.00000000000001421, 30.00000000000000355, 50.00000000000000000 ) ) ;
#5373=EDGE_LOOP ( 'NONE', ( #1493, #85, #5174, #1011, #4932 ) ) ;
#5388=ORIENTED_EDGE ( 'NONE', *, *, #1287, .T. ) ;
#5416=AXIS2_PLACEMENT_3D ( 'NONE', #5775, #234, #649 ) ;
#5419=LINE ( 'NONE', #3516, #4489 ) ;
#5461=VECTOR ( 'NONE', #2696, 1000.000000000000000 ) ;
#5477=CIRCLE ( 'NONE', #1495, 10.00000000000000178 ) ;
#5490=AXIS2_PLACEMENT_3D ( 'NONE', #1425, #4603, #1853 ) ;
#5511=DIRECTION ( 'NONE',  ( 0.000000000000000000, 1.000000000000000000, 0.000000000000000000 ) ) ;
#5542=EDGE_CURVE ( 'NONE', #111, #3568, #340, .T. ) ;
#5551=STYLED_ITEM ( 'NONE', ( #2910 ), #5861 ) ;
#5553=FACE_OUTER_BOUND ( 'NONE', #1018, .T. ) ;
#5556=VERTEX_POINT ( 'NONE', #4028 ) ;
#5571=ADVANCED_FACE ( 'NONE', ( #869 ), #1748, .T. ) ;
#5572=DIRECTION ( 'NONE',  ( 0.000000000000000000, -0.000000000000000000, 1.000000000000000000 ) ) ;
#5574=EDGE_CURVE ( 'NONE', #3549, #2954, #5419, .T. ) ;
#5578=AXIS2_PLACEMENT_3D ( 'NONE', #4757, #4219, #5572 ) ;
#5602=( LENGTH_UNIT ( ) NAMED_UNIT ( * ) SI_UNIT ( .MILLI., .METRE. ) );
#5630=CARTESIAN_POINT ( 'NONE',  ( -45.00000000000001421, 40.00000000000000000, -45.00000000000000000 ) ) ;
#5632=DIRECTION ( 'NONE',  ( 0.000000000000000000, 0.000000000000000000, -1.000000000000000000 ) ) ;
#5636=CARTESIAN_POINT ( 'NONE',  ( -45.00000000000001421, 40.00000000000000000, -50.00000000000000000 ) ) ;
#5664=DIRECTION ( 'NONE',  ( 1.000000000000000000, -0.000000000000000000, 0.000000000000000000 ) ) ;
#5668=SHAPE_REPRESENTATION_RELATIONSHIP ( 'NONE' , 'NONE' ,  #1113, #5861 ) ;
#5670=UNCERTAINTY_MEASURE_WITH_UNIT (LENGTH_MEASURE( 1.000000000000000082E-05 ), #4596, 'distance_accuracy_value', 'NONE');
#5688=ORIENTED_EDGE ( 'NONE', *, *, #5105, .T. ) ;
#5709=ORIENTED_EDGE ( 'NONE', *, *, #5949, .T. ) ;
#5711=LINE ( 'NONE', #4302, #1273 ) ;
#5713=CYLINDRICAL_SURFACE ( 'NONE', #3504, 10.00000000000000178 ) ;
#5733=CIRCLE ( 'NONE', #1368, 5.000000000000004441 ) ;
#5741=ORIENTED_EDGE ( 'NONE', *, *, #3702, .F. ) ;
#5746=ORIENTED_EDGE ( 'NONE', *, *, #3826, .T. ) ;
#5766=ORIENTED_EDGE ( 'NONE', *, *, #4249, .F. ) ;
#5771=ORIENTED_EDGE ( 'NONE', *, *, #1120, .F. ) ;
#5775=CARTESIAN_POINT ( 'NONE',  ( -45.00000000000001421, 30.00000000000000355, 45.00000000000000000 ) ) ;
#5797=AXIS2_PLACEMENT_3D ( 'NONE', #3215, #1349, #2229 ) ;
#5801=DIRECTION ( 'NONE',  ( -0.000000000000000000, -1.000000000000000000, -0.000000000000000000 ) ) ;
#5807=CYLINDRICAL_SURFACE ( 'NONE', #3126, 5.000000000000004441 ) ;
#5811=DIRECTION ( 'NONE',  ( 0.000000000000000000, 1.000000000000000000, 0.000000000000000000 ) ) ;
#5813=AXIS2_PLACEMENT_3D ( 'NONE', #5630, #3303, #996 ) ;
#5822=ORIENTED_EDGE ( 'NONE', *, *, #1723, .T. ) ;
#5826=AXIS2_PLACEMENT_3D ( 'NONE', #2613, #5801, #4478 ) ;
#5861=ADVANCED_BREP_SHAPE_REPRESENTATION ( '', ( #2182, #5080 ), #4776 ) ;
#5869=ORIENTED_EDGE ( 'NONE', *, *, #1756, .F. ) ;
#5874=CARTESIAN_POINT ( 'NONE',  ( -45.00000000000001421, 40.00000000000000000, 39.99999999999999289 ) ) ;
#5895=ORIENTED_EDGE ( 'NONE', *, *, #2791, .F. ) ;
#5901=ORIENTED_EDGE ( 'NONE', *, *, #3755, .T. ) ;
#5910=CIRCLE ( 'NONE', #1159, 10.00000000000000178 ) ;
#5913=LINE ( 'NONE', #3257, #2994 ) ;
#5918=ORIENTED_EDGE ( 'NONE', *, *, #1723, .F. ) ;
#5925=EDGE_LOOP ( 'NONE', ( #1257, #3803, #2033, #5135 ) ) ;
#5949=EDGE_CURVE ( 'NONE', #3109, #4600, #4288, .T. ) ;
#6000=COLOUR_RGB('Light Blue',0.38,0.62,0.78);
#6001=FILL_AREA_STYLE_COLOUR('',#6000);
#6002=FILL_AREA_STYLE('',(#6001));
#6003=SURFACE_STYLE_FILL_AREA(#6002);
#6004=SURFACE_SIDE_STYLE('',(#6003));
#6005=SURFACE_STYLE_USAGE(.BOTH.,#6004);
#6006=PRESENTATION_STYLE_ASSIGNMENT((#6005));
ENDSEC;
END-ISO-10303-21;
